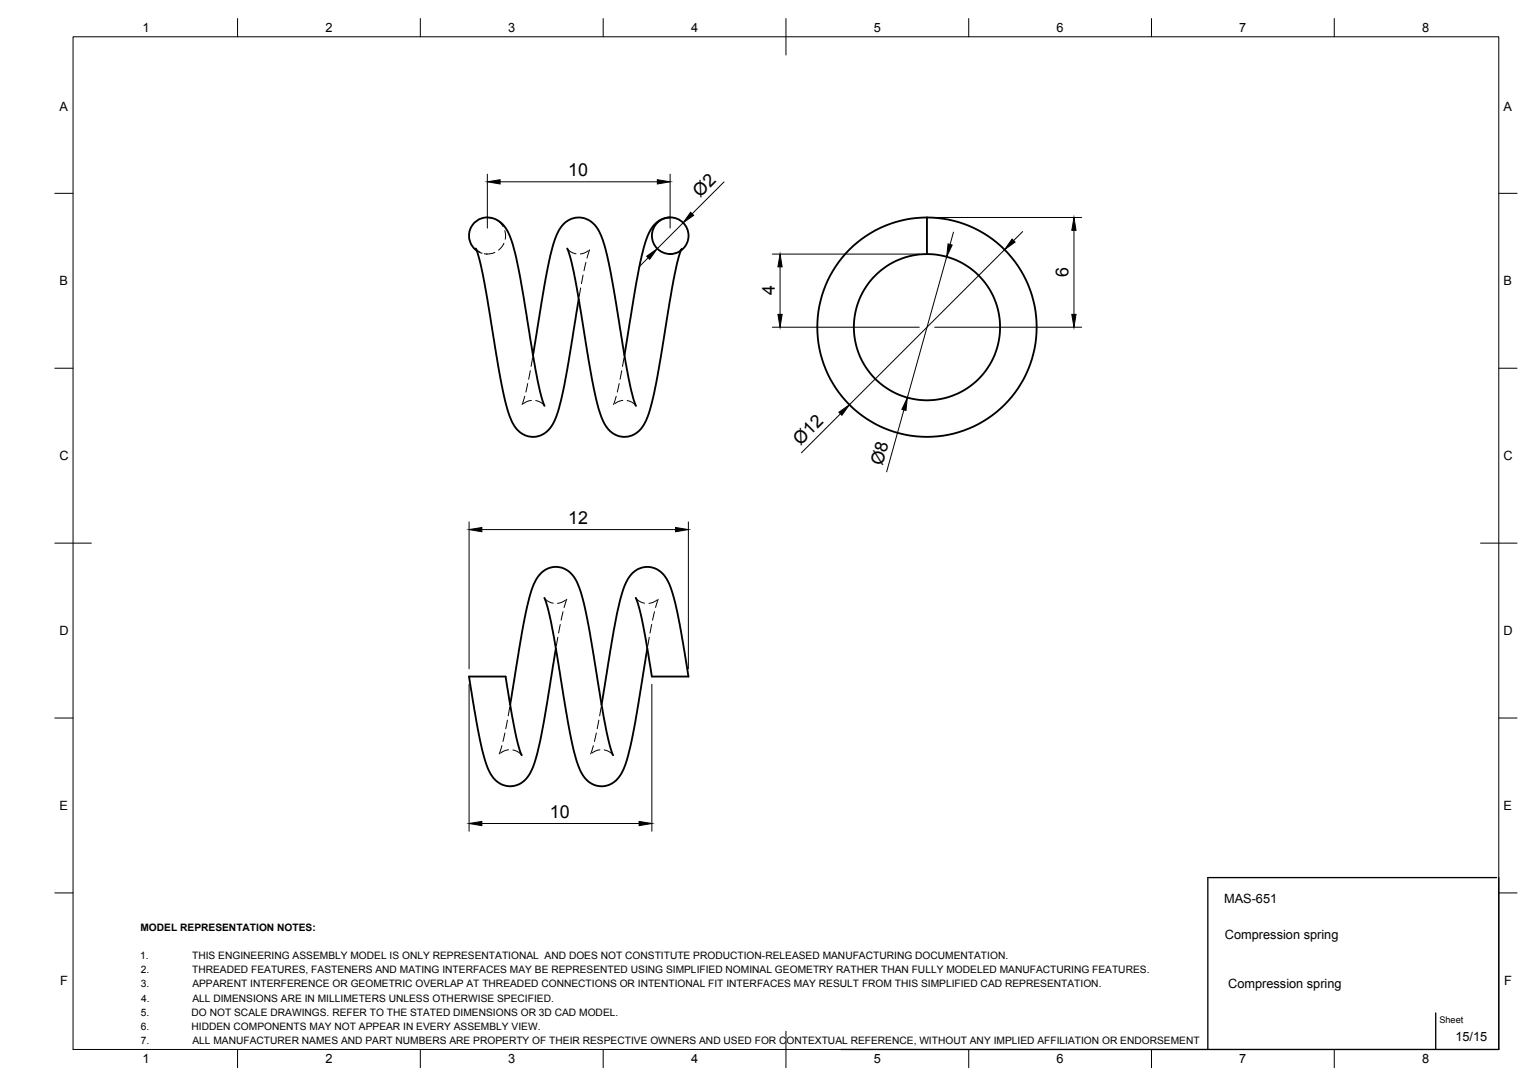
ISO-10303-21;
HEADER;
/* Generated by software containing ST-Developer
 * from STEP Tools, Inc. (www.steptools.com) 
 */

FILE_DESCRIPTION(
/* description */ ('Independent direct-acting normally-closed roller-plunger limit-switch
 CAD. Removable cover, insulated terminal supports, captured bus/conta
ct bridge, native Coil return spring, integral lower travel stop, reus
able instanced hardware and free roller. Manual geometric contact open
ing4mm; no snap-action/contact-force, electrical/current/voltage, envi
ronmental seal, safety-switch, wear, load or life certification. Exter
nal wiring and anchors omitted; fits and application engineering requi
red.'),
/* implementation_level */ '2;1');

FILE_NAME(
/* name */ 'Compression spring.step',
/* time_stamp */ '2026-11-08T07:32:43-08:00',
/* author */ (''),
/* organization */ (''),
/* preprocessor_version */ 'ST-DEVELOPER v20.2',
/* originating_system */ 'Autodesk Translation Framework v15.17.0.0',
/* authorisation */ '');

FILE_SCHEMA (('AUTOMOTIVE_DESIGN { 1 0 10303 214 3 1 1 }'));
ENDSEC;

DATA;
#10=MECHANICAL_DESIGN_GEOMETRIC_PRESENTATION_REPRESENTATION('',(#188),#36482);
#154=SHAPE_REPRESENTATION_RELATIONSHIP('SRR','None',#36567,#171);
#171=ADVANCED_BREP_SHAPE_REPRESENTATION('',(#205),#36477);
#188=STYLED_ITEM('',(#36660),#205);
#205=MANIFOLD_SOLID_BREP('Body1',#9779);
#228=B_SPLINE_SURFACE_WITH_KNOTS('',3,3,((#29315,#29316,#29317,#29318,#29319,
#29320,#29321,#29322,#29323,#29324,#29325,#29326,#29327,#29328,#29329,#29330,
#29331,#29332,#29333,#29334,#29335,#29336,#29337,#29338,#29339,#29340,#29341,
#29342,#29343),(#29344,#29345,#29346,#29347,#29348,#29349,#29350,#29351,
#29352,#29353,#29354,#29355,#29356,#29357,#29358,#29359,#29360,#29361,#29362,
#29363,#29364,#29365,#29366,#29367,#29368,#29369,#29370,#29371,#29372),
(#29373,#29374,#29375,#29376,#29377,#29378,#29379,#29380,#29381,#29382,
#29383,#29384,#29385,#29386,#29387,#29388,#29389,#29390,#29391,#29392,#29393,
#29394,#29395,#29396,#29397,#29398,#29399,#29400,#29401),(#29402,#29403,
#29404,#29405,#29406,#29407,#29408,#29409,#29410,#29411,#29412,#29413,#29414,
#29415,#29416,#29417,#29418,#29419,#29420,#29421,#29422,#29423,#29424,#29425,
#29426,#29427,#29428,#29429,#29430),(#29431,#29432,#29433,#29434,#29435,
#29436,#29437,#29438,#29439,#29440,#29441,#29442,#29443,#29444,#29445,#29446,
#29447,#29448,#29449,#29450,#29451,#29452,#29453,#29454,#29455,#29456,#29457,
#29458,#29459),(#29460,#29461,#29462,#29463,#29464,#29465,#29466,#29467,
#29468,#29469,#29470,#29471,#29472,#29473,#29474,#29475,#29476,#29477,#29478,
#29479,#29480,#29481,#29482,#29483,#29484,#29485,#29486,#29487,#29488),
(#29489,#29490,#29491,#29492,#29493,#29494,#29495,#29496,#29497,#29498,
#29499,#29500,#29501,#29502,#29503,#29504,#29505,#29506,#29507,#29508,#29509,
#29510,#29511,#29512,#29513,#29514,#29515,#29516,#29517),(#29518,#29519,
#29520,#29521,#29522,#29523,#29524,#29525,#29526,#29527,#29528,#29529,#29530,
#29531,#29532,#29533,#29534,#29535,#29536,#29537,#29538,#29539,#29540,#29541,
#29542,#29543,#29544,#29545,#29546),(#29547,#29548,#29549,#29550,#29551,
#29552,#29553,#29554,#29555,#29556,#29557,#29558,#29559,#29560,#29561,#29562,
#29563,#29564,#29565,#29566,#29567,#29568,#29569,#29570,#29571,#29572,#29573,
#29574,#29575),(#29576,#29577,#29578,#29579,#29580,#29581,#29582,#29583,
#29584,#29585,#29586,#29587,#29588,#29589,#29590,#29591,#29592,#29593,#29594,
#29595,#29596,#29597,#29598,#29599,#29600,#29601,#29602,#29603,#29604)),
 .UNSPECIFIED.,.T.,.F.,.F.,(4,1,1,1,1,1,1,4),(4,1,1,1,1,1,1,1,1,1,1,1,1,
1,1,1,1,1,1,1,1,1,1,1,1,1,4),(-3.14159265358979,-2.24399475256414,-1.34639685153848,
-0.448798950512828,0.448798950512828,1.34639685153848,2.24399475256414,
3.14159265358979),(0.,0.483321946706122,0.966643893412244,1.44996584011837,
1.93328778682449,2.41660973353061,2.89993168023673,3.38325362694285,3.86657557364898,
4.3498975203551,4.83321946706122,5.31654141376734,5.79986336047346,6.28318530717959,
6.76650725388571,7.24982920059183,7.73315114729795,8.21647309400407,8.6997950407102,
9.18311698741632,9.66643893412244,10.1497608808286,10.6330828275347,11.1164047742408,
11.5997267209469,12.083048667653,12.5663706143592),.UNSPECIFIED.);
#405=PLANE('',#10494);
#406=PLANE('',#10495);
#834=FACE_OUTER_BOUND('',#1431,.T.);
#835=FACE_OUTER_BOUND('',#1432,.T.);
#836=FACE_OUTER_BOUND('',#1433,.T.);
#1431=EDGE_LOOP('',(#8098,#8099,#8100,#8101));
#1432=EDGE_LOOP('',(#8102));
#1433=EDGE_LOOP('',(#8103));
#1711=CIRCLE('',#10492,0.1);
#1712=CIRCLE('',#10493,0.1);
#2241=B_SPLINE_CURVE_WITH_KNOTS('',3,(#29608,#29609,#29610,#29611,#29612,
#29613,#29614,#29615,#29616,#29617,#29618,#29619,#29620,#29621,#29622,#29623,
#29624,#29625,#29626,#29627,#29628,#29629,#29630,#29631,#29632,#29633,#29634,
#29635,#29636),.UNSPECIFIED.,.F.,.F.,(4,1,1,1,1,1,1,1,1,1,1,1,1,1,1,1,1,
1,1,1,1,1,1,1,1,1,4),(0.,0.483321946706122,0.966643893412244,1.44996584011837,
1.93328778682449,2.41660973353061,2.89993168023673,3.38325362694285,3.86657557364898,
4.3498975203551,4.83321946706122,5.31654141376734,5.79986336047346,6.28318530717959,
6.76650725388571,7.24982920059183,7.73315114729795,8.21647309400407,8.6997950407102,
9.18311698741632,9.66643893412244,10.1497608808286,10.6330828275347,11.1164047742408,
11.5997267209469,12.083048667653,12.5663706143592),.UNSPECIFIED.);
#4295=VERTEX_POINT('',#29605);
#4296=VERTEX_POINT('',#29607);
#5605=EDGE_CURVE('',#4295,#4295,#1711,.T.);
#5606=EDGE_CURVE('',#4295,#4296,#2241,.T.);
#5607=EDGE_CURVE('',#4296,#4296,#1712,.T.);
#8098=ORIENTED_EDGE('',*,*,#5605,.T.);
#8099=ORIENTED_EDGE('',*,*,#5606,.T.);
#8100=ORIENTED_EDGE('',*,*,#5607,.F.);
#8101=ORIENTED_EDGE('',*,*,#5606,.F.);
#8102=ORIENTED_EDGE('',*,*,#5607,.T.);
#8103=ORIENTED_EDGE('',*,*,#5605,.F.);
#9624=ADVANCED_FACE('',(#834),#228,.T.);
#9625=ADVANCED_FACE('',(#835),#405,.F.);
#9626=ADVANCED_FACE('',(#836),#406,.T.);
#9779=CLOSED_SHELL('',(#9624,#9625,#9626));
#10491=AXIS2_PLACEMENT_3D('',#29314,#12152,#12153);
#10492=AXIS2_PLACEMENT_3D('',#29606,#12154,#12155);
#10493=AXIS2_PLACEMENT_3D('',#29637,#12156,#12157);
#10494=AXIS2_PLACEMENT_3D('',#29638,#12158,#12159);
#10495=AXIS2_PLACEMENT_3D('',#29639,#12160,#12161);
#12152=DIRECTION('axis',(0.,0.,1.));
#12153=DIRECTION('refdir',(1.,0.,0.));
#12154=DIRECTION('center_axis',(0.,0.,-1.));
#12155=DIRECTION('ref_axis',(-1.,0.,0.));
#12156=DIRECTION('center_axis',(4.89858719658941E-16,0.,-1.));
#12157=DIRECTION('ref_axis',(-1.,0.,-4.89858719658941E-16));
#12158=DIRECTION('center_axis',(-4.89858719658941E-16,0.,1.));
#12159=DIRECTION('ref_axis',(1.,0.,4.89858719658941E-16));
#12160=DIRECTION('center_axis',(0.,0.,1.));
#12161=DIRECTION('ref_axis',(1.,0.,0.));
#29314=CARTESIAN_POINT('',(0.,0.,0.));
#29315=CARTESIAN_POINT('Ctrl Pts',(0.6,-1.22464679914735E-17,0.));
#29316=CARTESIAN_POINT('Ctrl Pts',(0.6,0.0128205128205128,-0.0966643893412244));
#29317=CARTESIAN_POINT('Ctrl Pts',(0.552422075024677,0.0384615384615385,
-0.289907779312461));
#29318=CARTESIAN_POINT('Ctrl Pts',(0.354387423761003,0.0769230769230769,
-0.513439446520879));
#29319=CARTESIAN_POINT('Ctrl Pts',(0.0752027553952744,0.115384615384615,
-0.619312950390957));
#29320=CARTESIAN_POINT('Ctrl Pts',(-0.221227750860346,0.153846153846154,
-0.583326335743102));
#29321=CARTESIAN_POINT('Ctrl Pts',(-0.466969125257516,0.192307692307692,
-0.413698471057249));
#29322=CARTESIAN_POINT('Ctrl Pts',(-0.605737625154647,0.230769230769231,
-0.149301246402526));
#29323=CARTESIAN_POINT('Ctrl Pts',(-0.605736940333524,0.269230769230769,
0.14930101675222));
#29324=CARTESIAN_POINT('Ctrl Pts',(-0.466970187413293,0.307692307692308,
0.413699286558057));
#29325=CARTESIAN_POINT('Ctrl Pts',(-0.221225725123394,0.346153846153846,
0.583324484886018));
#29326=CARTESIAN_POINT('Ctrl Pts',(0.0751986583056162,0.384615384615385,
0.619316856641734));
#29327=CARTESIAN_POINT('Ctrl Pts',(0.354396045955746,0.423076923076923,
0.513431304005641));
#29328=CARTESIAN_POINT('Ctrl Pts',(0.55240551470084,0.461538461538462,0.289924779022985));
#29329=CARTESIAN_POINT('Ctrl Pts',(0.623865568763842,0.5,3.99584594159288E-16));
#29330=CARTESIAN_POINT('Ctrl Pts',(0.552405514700841,0.538461538461539,
-0.289924779022984));
#29331=CARTESIAN_POINT('Ctrl Pts',(0.354396045955747,0.576923076923077,
-0.513431304005641));
#29332=CARTESIAN_POINT('Ctrl Pts',(0.0751986583056171,0.615384615384616,
-0.619316856641735));
#29333=CARTESIAN_POINT('Ctrl Pts',(-0.221225725123393,0.653846153846154,
-0.583324484886017));
#29334=CARTESIAN_POINT('Ctrl Pts',(-0.466970187413293,0.692307692307693,
-0.413699286558058));
#29335=CARTESIAN_POINT('Ctrl Pts',(-0.605736940333523,0.730769230769231,
-0.149301016752221));
#29336=CARTESIAN_POINT('Ctrl Pts',(-0.605737625154647,0.769230769230769,
0.149301246402525));
#29337=CARTESIAN_POINT('Ctrl Pts',(-0.466969125257516,0.807692307692308,
0.41369847105725));
#29338=CARTESIAN_POINT('Ctrl Pts',(-0.221227750860347,0.846153846153846,
0.583326335743102));
#29339=CARTESIAN_POINT('Ctrl Pts',(0.0752027553952735,0.884615384615385,
0.619312950390957));
#29340=CARTESIAN_POINT('Ctrl Pts',(0.354387423761003,0.923076923076923,
0.513439446520879));
#29341=CARTESIAN_POINT('Ctrl Pts',(0.552422075024676,0.961538461538462,
0.289907779312462));
#29342=CARTESIAN_POINT('Ctrl Pts',(0.6,0.987179487179487,0.096664389341225));
#29343=CARTESIAN_POINT('Ctrl Pts',(0.6,1.,2.93915231795365E-16));
#29344=CARTESIAN_POINT('Ctrl Pts',(0.6,-0.0299199300341885,0.));
#29345=CARTESIAN_POINT('Ctrl Pts',(0.6,-0.0170994172136757,-0.09670823080664));
#29346=CARTESIAN_POINT('Ctrl Pts',(0.552433668035603,0.00854160842734991,
-0.289889597147613));
#29347=CARTESIAN_POINT('Ctrl Pts',(0.354391049739123,0.0470031468888885,
-0.513458052176708));
#29348=CARTESIAN_POINT('Ctrl Pts',(0.0752046939357531,0.0854646853504268,
-0.619317061421753));
#29349=CARTESIAN_POINT('Ctrl Pts',(-0.221231470738224,0.123926223811965,
-0.583337632633336));
#29350=CARTESIAN_POINT('Ctrl Pts',(-0.466975962510102,0.162387762273504,
-0.413703477287484));
#29351=CARTESIAN_POINT('Ctrl Pts',(-0.605746831003298,0.200849300735043,
-0.149304082326356));
#29352=CARTESIAN_POINT('Ctrl Pts',(-0.605746010438017,0.239310839196581,
0.149303548319889));
#29353=CARTESIAN_POINT('Ctrl Pts',(-0.466977235204714,0.277772377658119,
0.413705373558643));
#29354=CARTESIAN_POINT('Ctrl Pts',(-0.221229043462903,0.316233916119658,
0.58333332852287));
#29355=CARTESIAN_POINT('Ctrl Pts',(0.0751997847274774,0.354695454581196,
0.619326143478273));
#29356=CARTESIAN_POINT('Ctrl Pts',(0.35440138101164,0.393156993042734,0.513439044221362));
#29357=CARTESIAN_POINT('Ctrl Pts',(0.552413825150628,0.431618531504273,
0.289929135658685));
#29358=CARTESIAN_POINT('Ctrl Pts',(0.623874957033007,0.470080069965812,
3.99584594159288E-16));
#29359=CARTESIAN_POINT('Ctrl Pts',(0.552413825150628,0.50854160842735,-0.289929135658685));
#29360=CARTESIAN_POINT('Ctrl Pts',(0.354401381011641,0.547003146888889,
-0.513439044221361));
#29361=CARTESIAN_POINT('Ctrl Pts',(0.0751997847274784,0.585464685350427,
-0.619326143478273));
#29362=CARTESIAN_POINT('Ctrl Pts',(-0.221229043462903,0.623926223811966,
-0.583333328522871));
#29363=CARTESIAN_POINT('Ctrl Pts',(-0.466977235204713,0.662387762273504,
-0.413705373558643));
#29364=CARTESIAN_POINT('Ctrl Pts',(-0.605746010438017,0.700849300735043,
-0.14930354831989));
#29365=CARTESIAN_POINT('Ctrl Pts',(-0.605746831003298,0.73931083919658,
0.149304082326356));
#29366=CARTESIAN_POINT('Ctrl Pts',(-0.466975962510103,0.77777237765812,
0.413703477287484));
#29367=CARTESIAN_POINT('Ctrl Pts',(-0.221231470738224,0.816233916119658,
0.583337632633336));
#29368=CARTESIAN_POINT('Ctrl Pts',(0.0752046939357522,0.854695454581196,
0.619317061421752));
#29369=CARTESIAN_POINT('Ctrl Pts',(0.354391049739122,0.893156993042734,
0.513458052176709));
#29370=CARTESIAN_POINT('Ctrl Pts',(0.552433668035603,0.931618531504273,
0.289889597147614));
#29371=CARTESIAN_POINT('Ctrl Pts',(0.6,0.957259557145299,0.0967082308066405));
#29372=CARTESIAN_POINT('Ctrl Pts',(0.6,0.970080069965812,2.93915231795365E-16));
#29373=CARTESIAN_POINT('Ctrl Pts',(0.57140278473399,-0.0895099491231781,
0.));
#29374=CARTESIAN_POINT('Ctrl Pts',(0.57140278473399,-0.0766894363026653,
-0.0920388134316465));
#29375=CARTESIAN_POINT('Ctrl Pts',(0.526087666325587,-0.0510484106616395,
-0.27609779977643));
#29376=CARTESIAN_POINT('Ctrl Pts',(0.337495083246531,-0.0125868722001011,
-0.488960092834314));
#29377=CARTESIAN_POINT('Ctrl Pts',(0.071617628135789,0.0258746662614374,
-0.589793519606227));
#29378=CARTESIAN_POINT('Ctrl Pts',(-0.210682030750213,0.064336204722976,
-0.555519091361673));
#29379=CARTESIAN_POINT('Ctrl Pts',(-0.444709568341539,0.102797743184514,
-0.393978668020424));
#29380=CARTESIAN_POINT('Ctrl Pts',(-0.57686308879389,0.141259281646053,
-0.142184059267368));
#29381=CARTESIAN_POINT('Ctrl Pts',(-0.576862493445414,0.179720820107591,
0.142183967988976));
#29382=CARTESIAN_POINT('Ctrl Pts',(-0.444710491725475,0.21818235856913,
0.39397899216129));
#29383=CARTESIAN_POINT('Ctrl Pts',(-0.21068026967806,0.256643897030668,
0.555518355836033));
#29384=CARTESIAN_POINT('Ctrl Pts',(0.0716140663354809,0.295105435492207,
0.589795072696736));
#29385=CARTESIAN_POINT('Ctrl Pts',(0.337502578941879,0.333566973953745,
0.488956887495931));
#29386=CARTESIAN_POINT('Ctrl Pts',(0.526073269626597,0.372028512415283,
0.276104552814102));
#29387=CARTESIAN_POINT('Ctrl Pts',(0.59412694151864,0.410490050876822,3.42501080707961E-16));
#29388=CARTESIAN_POINT('Ctrl Pts',(0.526073269626597,0.448951589338361,
-0.276104552814101));
#29389=CARTESIAN_POINT('Ctrl Pts',(0.33750257894188,0.487413127799899,-0.488956887495931));
#29390=CARTESIAN_POINT('Ctrl Pts',(0.0716140663354816,0.525874666261437,
-0.589795072696736));
#29391=CARTESIAN_POINT('Ctrl Pts',(-0.21068026967806,0.564336204722976,
-0.555518355836033));
#29392=CARTESIAN_POINT('Ctrl Pts',(-0.444710491725474,0.602797743184515,
-0.393978992161291));
#29393=CARTESIAN_POINT('Ctrl Pts',(-0.576862493445414,0.641259281646054,
-0.142183967988976));
#29394=CARTESIAN_POINT('Ctrl Pts',(-0.576863088793891,0.679720820107591,
0.142184059267367));
#29395=CARTESIAN_POINT('Ctrl Pts',(-0.44470956834154,0.718182358569131,
0.393978668020424));
#29396=CARTESIAN_POINT('Ctrl Pts',(-0.210682030750213,0.756643897030668,
0.555519091361672));
#29397=CARTESIAN_POINT('Ctrl Pts',(0.0716176281357881,0.795105435492208,
0.589793519606227));
#29398=CARTESIAN_POINT('Ctrl Pts',(0.33749508324653,0.833566973953744,0.488960092834314));
#29399=CARTESIAN_POINT('Ctrl Pts',(0.526087666325587,0.872028512415284,
0.276097799776431));
#29400=CARTESIAN_POINT('Ctrl Pts',(0.57140278473399,0.89766953805631,0.092038813431647));
#29401=CARTESIAN_POINT('Ctrl Pts',(0.57140278473399,0.910490050876822,2.79906636539346E-16));
#29402=CARTESIAN_POINT('Ctrl Pts',(0.474553946216323,-0.111561765583155,
0.));
#29403=CARTESIAN_POINT('Ctrl Pts',(0.474553946216323,-0.0987412527626418,
-0.0764564796257483));
#29404=CARTESIAN_POINT('Ctrl Pts',(0.436924085441389,-0.0731002271216164,
-0.229293819423993));
#29405=CARTESIAN_POINT('Ctrl Pts',(0.28029344651323,-0.0346386886600778,
-0.406092197111352));
#29406=CARTESIAN_POINT('Ctrl Pts',(0.0594797119051372,0.00382284980146056,
-0.489829229563544));
#29407=CARTESIAN_POINT('Ctrl Pts',(-0.174974371163627,0.0422843882629991,
-0.461366967583472));
#29408=CARTESIAN_POINT('Ctrl Pts',(-0.369337104437002,0.0807459267245375,
-0.327204006955578));
#29409=CARTESIAN_POINT('Ctrl Pts',(-0.479092464392592,0.119207465186076,
-0.118085979220413));
#29410=CARTESIAN_POINT('Ctrl Pts',(-0.479091915422023,0.157669003647615,
0.118085781150671));
#29411=CARTESIAN_POINT('Ctrl Pts',(-0.369337955888923,0.196130542109153,
0.327204710311264));
#29412=CARTESIAN_POINT('Ctrl Pts',(-0.17497274727977,0.234592080570691,
0.461365371232019));
#29413=CARTESIAN_POINT('Ctrl Pts',(0.0594764275706395,0.27305361903223,
0.489832598580241));
#29414=CARTESIAN_POINT('Ctrl Pts',(0.280300358290614,0.311515157493768,
0.406085170317839));
#29415=CARTESIAN_POINT('Ctrl Pts',(0.436910810251582,0.349976695955307,
0.229308481892446));
#29416=CARTESIAN_POINT('Ctrl Pts',(0.493430286203431,0.388438234416845,
3.28230202345129E-16));
#29417=CARTESIAN_POINT('Ctrl Pts',(0.436910810251583,0.426899772878384,
-0.229308481892445));
#29418=CARTESIAN_POINT('Ctrl Pts',(0.280300358290614,0.465361311339922,
-0.406085170317838));
#29419=CARTESIAN_POINT('Ctrl Pts',(0.0594764275706403,0.503822849801461,
-0.489832598580241));
#29420=CARTESIAN_POINT('Ctrl Pts',(-0.17497274727977,0.542284388262999,
-0.461365371232019));
#29421=CARTESIAN_POINT('Ctrl Pts',(-0.369337955888923,0.580745926724537,
-0.327204710311264));
#29422=CARTESIAN_POINT('Ctrl Pts',(-0.479091915422023,0.619207465186076,
-0.118085781150672));
#29423=CARTESIAN_POINT('Ctrl Pts',(-0.479092464392592,0.657669003647615,
0.118085979220413));
#29424=CARTESIAN_POINT('Ctrl Pts',(-0.369337104437003,0.696130542109153,
0.327204006955579));
#29425=CARTESIAN_POINT('Ctrl Pts',(-0.174974371163627,0.734592080570691,
0.461366967583471));
#29426=CARTESIAN_POINT('Ctrl Pts',(0.0594797119051365,0.773053619032229,
0.489829229563544));
#29427=CARTESIAN_POINT('Ctrl Pts',(0.280293446513229,0.811515157493768,
0.406092197111352));
#29428=CARTESIAN_POINT('Ctrl Pts',(0.436924085441388,0.849976695955308,
0.229293819423994));
#29429=CARTESIAN_POINT('Ctrl Pts',(0.474553946216323,0.875617721596332,
0.0764564796257487));
#29430=CARTESIAN_POINT('Ctrl Pts',(0.474553946216323,0.888438234416845,
2.32464388502626E-16));
#29431=CARTESIAN_POINT('Ctrl Pts',(0.396775149169774,-0.0496835058675068,
0.));
#29432=CARTESIAN_POINT('Ctrl Pts',(0.396775149169774,-0.036862993046994,
-0.0639325270983766));
#29433=CARTESIAN_POINT('Ctrl Pts',(0.365314671027668,-0.0112219674059683,
-0.19170987675844));
#29434=CARTESIAN_POINT('Ctrl Pts',(0.23435429480531,0.0272395710555702,
-0.339537237215488));
#29435=CARTESIAN_POINT('Ctrl Pts',(0.0497313786444746,0.0657011095171087,
-0.409547504928549));
#29436=CARTESIAN_POINT('Ctrl Pts',(-0.146296899267444,0.104162647978647,
-0.385751347000212));
#29437=CARTESIAN_POINT('Ctrl Pts',(-0.308804333876165,0.142624186440185,
-0.273576498871778));
#29438=CARTESIAN_POINT('Ctrl Pts',(-0.400571315183775,0.181085724901724,
-0.0987322989296554));
#29439=CARTESIAN_POINT('Ctrl Pts',(-0.400570833992816,0.219547263363262,
0.098732083557009));
#29440=CARTESIAN_POINT('Ctrl Pts',(-0.308805080202088,0.258008801824801,
0.273577263668698));
#29441=CARTESIAN_POINT('Ctrl Pts',(-0.146295475879243,0.296470340286339,
0.385749611149152));
#29442=CARTESIAN_POINT('Ctrl Pts',(0.0497284998160722,0.334931878747878,
0.409551168080821));
#29443=CARTESIAN_POINT('Ctrl Pts',(0.234360353208027,0.373393417209416,
0.339529585460424));
#29444=CARTESIAN_POINT('Ctrl Pts',(0.365303034882358,0.411854955670955,
0.19172582146083));
#29445=CARTESIAN_POINT('Ctrl Pts',(0.412559215796984,0.450316494132494,
2.28334053805307E-16));
#29446=CARTESIAN_POINT('Ctrl Pts',(0.365303034882358,0.488778032594032,
-0.191725821460829));
#29447=CARTESIAN_POINT('Ctrl Pts',(0.234360353208027,0.52723957105557,-0.339529585460423));
#29448=CARTESIAN_POINT('Ctrl Pts',(0.049728499816073,0.565701109517109,
-0.409551168080821));
#29449=CARTESIAN_POINT('Ctrl Pts',(-0.146295475879243,0.604162647978647,
-0.385749611149151));
#29450=CARTESIAN_POINT('Ctrl Pts',(-0.308805080202087,0.642624186440186,
-0.273577263668699));
#29451=CARTESIAN_POINT('Ctrl Pts',(-0.400570833992816,0.681085724901724,
-0.0987320835570092));
#29452=CARTESIAN_POINT('Ctrl Pts',(-0.400571315183774,0.719547263363262,
0.0987322989296545));
#29453=CARTESIAN_POINT('Ctrl Pts',(-0.308804333876166,0.758008801824802,
0.273576498871779));
#29454=CARTESIAN_POINT('Ctrl Pts',(-0.146296899267444,0.79647034028634,
0.385751347000211));
#29455=CARTESIAN_POINT('Ctrl Pts',(0.0497313786444738,0.834931878747878,
0.409547504928549));
#29456=CARTESIAN_POINT('Ctrl Pts',(0.234354294805309,0.873393417209416,
0.339537237215489));
#29457=CARTESIAN_POINT('Ctrl Pts',(0.365314671027668,0.911854955670954,
0.191709876758441));
#29458=CARTESIAN_POINT('Ctrl Pts',(0.396775149169774,0.937495981311981,
0.0639325270983769));
#29459=CARTESIAN_POINT('Ctrl Pts',(0.396775149169774,0.950316494132494,
1.94363766564791E-16));
#29460=CARTESIAN_POINT('Ctrl Pts',(0.396939270424005,0.0496169828764393,
0.));
#29461=CARTESIAN_POINT('Ctrl Pts',(0.396939270424005,0.0624374956969522,
-0.0639374232798038));
#29462=CARTESIAN_POINT('Ctrl Pts',(0.36546008089603,0.0880785213379777,
-0.191798112042878));
#29463=CARTESIAN_POINT('Ctrl Pts',(0.234449450409805,0.126540059799516,
-0.339668537739251));
#29464=CARTESIAN_POINT('Ctrl Pts',(0.049750996607657,0.165001598261055,
-0.409714888680431));
#29465=CARTESIAN_POINT('Ctrl Pts',(-0.146355584839357,0.203463136722593,
-0.385905355800823));
#29466=CARTESIAN_POINT('Ctrl Pts',(-0.308928706451725,0.241924675184131,
-0.273687199853259));
#29467=CARTESIAN_POINT('Ctrl Pts',(-0.400732481863726,0.28038621364567,
-0.0987717444550605));
#29468=CARTESIAN_POINT('Ctrl Pts',(-0.400732067194017,0.318847752107208,
0.0987716785889419));
#29469=CARTESIAN_POINT('Ctrl Pts',(-0.308929349603364,0.357309290568747,
0.273687433751705));
#29470=CARTESIAN_POINT('Ctrl Pts',(-0.146354358224513,0.395770829030285,
0.385904825042549));
#29471=CARTESIAN_POINT('Ctrl Pts',(0.0497485157569321,0.434232367491824,
0.40971600936184));
#29472=CARTESIAN_POINT('Ctrl Pts',(0.234454671281171,0.472693905953362,
0.339666223345759));
#29473=CARTESIAN_POINT('Ctrl Pts',(0.365450053365557,0.511155444414901,
0.191802985182395));
#29474=CARTESIAN_POINT('Ctrl Pts',(0.412725251465001,0.549616982876439,
3.13959323982298E-16));
#29475=CARTESIAN_POINT('Ctrl Pts',(0.365450053365557,0.588078521337977,
-0.191802985182395));
#29476=CARTESIAN_POINT('Ctrl Pts',(0.234454671281172,0.626540059799516,
-0.339666223345758));
#29477=CARTESIAN_POINT('Ctrl Pts',(0.0497485157569325,0.665001598261056,
-0.409716009361841));
#29478=CARTESIAN_POINT('Ctrl Pts',(-0.146354358224513,0.703463136722593,
-0.385904825042548));
#29479=CARTESIAN_POINT('Ctrl Pts',(-0.308929349603364,0.741924675184131,
-0.273687433751706));
#29480=CARTESIAN_POINT('Ctrl Pts',(-0.400732067194016,0.78038621364567,
-0.0987716785889423));
#29481=CARTESIAN_POINT('Ctrl Pts',(-0.400732481863727,0.818847752107209,
0.09877174445506));
#29482=CARTESIAN_POINT('Ctrl Pts',(-0.308928706451726,0.857309290568746,
0.273687199853259));
#29483=CARTESIAN_POINT('Ctrl Pts',(-0.146355584839357,0.895770829030286,
0.385905355800823));
#29484=CARTESIAN_POINT('Ctrl Pts',(0.0497509966076566,0.934232367491823,
0.409714888680431));
#29485=CARTESIAN_POINT('Ctrl Pts',(0.234449450409805,0.972693905953362,
0.339668537739251));
#29486=CARTESIAN_POINT('Ctrl Pts',(0.36546008089603,1.0111554444149,0.191798112042878));
#29487=CARTESIAN_POINT('Ctrl Pts',(0.396939270424005,1.03679647005593,0.0639374232798042));
#29488=CARTESIAN_POINT('Ctrl Pts',(0.396939270424005,1.04961698287644,1.94444162792257E-16));
#29489=CARTESIAN_POINT('Ctrl Pts',(0.474480121999477,0.111725197096412,
0.));
#29490=CARTESIAN_POINT('Ctrl Pts',(0.474480121999477,0.124545709916925,
-0.0764586335789696));
#29491=CARTESIAN_POINT('Ctrl Pts',(0.436859829833703,0.150186735557951,
-0.229252323181468));
#29492=CARTESIAN_POINT('Ctrl Pts',(0.28025100438353,0.188648274019489,-0.406034984914813));
#29493=CARTESIAN_POINT('Ctrl Pts',(0.0594710800733114,0.227109812481028,
-0.489754346320688));
#29494=CARTESIAN_POINT('Ctrl Pts',(-0.174948343135337,0.265571350942566,
-0.461298814622112));
#29495=CARTESIAN_POINT('Ctrl Pts',(-0.369281839162736,0.304032889404105,
-0.327154709430175));
#29496=CARTESIAN_POINT('Ctrl Pts',(-0.479020883931678,0.342494427865643,
-0.118068517820842));
#29497=CARTESIAN_POINT('Ctrl Pts',(-0.47902029155056,0.380955966327182,
0.118068222258303));
#29498=CARTESIAN_POINT('Ctrl Pts',(-0.369282757944306,0.41941750478872,
0.327155758983302));
#29499=CARTESIAN_POINT('Ctrl Pts',(-0.17494659084079,0.457879043250258,
0.461296432432969));
#29500=CARTESIAN_POINT('Ctrl Pts',(0.0594675360258692,0.496340581711797,
0.489759373275717));
#29501=CARTESIAN_POINT('Ctrl Pts',(0.280258462718537,0.534802120173335,
0.406024477645537));
#29502=CARTESIAN_POINT('Ctrl Pts',(0.436845504891309,0.573263658634874,
0.22927420538536));
#29503=CARTESIAN_POINT('Ctrl Pts',(0.493356533724516,0.611725197096412,
3.99584594159288E-16));
#29504=CARTESIAN_POINT('Ctrl Pts',(0.43684550489131,0.650186735557951,-0.229274205385359));
#29505=CARTESIAN_POINT('Ctrl Pts',(0.280258462718538,0.688648274019488,
-0.406024477645536));
#29506=CARTESIAN_POINT('Ctrl Pts',(0.0594675360258697,0.727109812481028,
-0.489759373275717));
#29507=CARTESIAN_POINT('Ctrl Pts',(-0.174946590840789,0.765571350942565,
-0.461296432432969));
#29508=CARTESIAN_POINT('Ctrl Pts',(-0.369282757944306,0.804032889404106,
-0.327155758983302));
#29509=CARTESIAN_POINT('Ctrl Pts',(-0.47902029155056,0.842494427865642,
-0.118068222258304));
#29510=CARTESIAN_POINT('Ctrl Pts',(-0.479020883931677,0.880955966327181,
0.118068517820842));
#29511=CARTESIAN_POINT('Ctrl Pts',(-0.369281839162738,0.91941750478872,
0.327154709430175));
#29512=CARTESIAN_POINT('Ctrl Pts',(-0.174948343135337,0.957879043250258,
0.461298814622112));
#29513=CARTESIAN_POINT('Ctrl Pts',(0.0594710800733105,0.996340581711796,
0.489754346320688));
#29514=CARTESIAN_POINT('Ctrl Pts',(0.28025100438353,1.03480212017334,0.406034984914813));
#29515=CARTESIAN_POINT('Ctrl Pts',(0.436859829833702,1.07326365863487,0.229252323181468));
#29516=CARTESIAN_POINT('Ctrl Pts',(0.474480121999477,1.0989046842759,0.0764586335789701));
#29517=CARTESIAN_POINT('Ctrl Pts',(0.474480121999477,1.11172519709641,2.32428225066282E-16));
#29518=CARTESIAN_POINT('Ctrl Pts',(0.571396374369977,0.0893939875669938,
0.));
#29519=CARTESIAN_POINT('Ctrl Pts',(0.571396374369977,0.102214500387507,
-0.0920304506152003));
#29520=CARTESIAN_POINT('Ctrl Pts',(0.526079825991483,0.127855526028532,
-0.27609774238039));
#29521=CARTESIAN_POINT('Ctrl Pts',(0.337490690748289,0.166317064490071,
-0.488951496511335));
#29522=CARTESIAN_POINT('Ctrl Pts',(0.0716165005604001,0.204778602951609,
-0.589786215561319));
#29523=CARTESIAN_POINT('Ctrl Pts',(-0.210679045222389,0.243240141413148,
-0.555510970358107));
#29524=CARTESIAN_POINT('Ctrl Pts',(-0.444703436119133,0.281701679874686,
-0.393973411075695));
#29525=CARTESIAN_POINT('Ctrl Pts',(-0.576855077960488,0.320163218336225,
-0.142181989990421));
#29526=CARTESIAN_POINT('Ctrl Pts',(-0.576854505315029,0.358624756797763,
0.142181949601214));
#29527=CARTESIAN_POINT('Ctrl Pts',(-0.444704324290748,0.397086295259301,
0.393973554508792));
#29528=CARTESIAN_POINT('Ctrl Pts',(-0.210677351306959,0.43554783372084,
0.555510645023163));
#29529=CARTESIAN_POINT('Ctrl Pts',(0.0716130745857797,0.474009372182378,
0.589786903242894));
#29530=CARTESIAN_POINT('Ctrl Pts',(0.337497900602802,0.512470910643917,
0.48895010790376));
#29531=CARTESIAN_POINT('Ctrl Pts',(0.526065978296192,0.550932449105455,
0.276100726868827));
#29532=CARTESIAN_POINT('Ctrl Pts',(0.594118706507634,0.589393987566993,
4.28126350884951E-16));
#29533=CARTESIAN_POINT('Ctrl Pts',(0.526065978296193,0.627855526028533,
-0.276100726868826));
#29534=CARTESIAN_POINT('Ctrl Pts',(0.337497900602802,0.66631706449007,-0.48895010790376));
#29535=CARTESIAN_POINT('Ctrl Pts',(0.0716130745857805,0.70477860295161,
-0.589786903242894));
#29536=CARTESIAN_POINT('Ctrl Pts',(-0.210677351306959,0.743240141413148,
-0.555510645023163));
#29537=CARTESIAN_POINT('Ctrl Pts',(-0.444704324290748,0.781701679874686,
-0.393973554508792));
#29538=CARTESIAN_POINT('Ctrl Pts',(-0.576854505315029,0.820163218336225,
-0.142181949601214));
#29539=CARTESIAN_POINT('Ctrl Pts',(-0.576855077960488,0.858624756797763,
0.14218198999042));
#29540=CARTESIAN_POINT('Ctrl Pts',(-0.444703436119134,0.897086295259303,
0.393973411075695));
#29541=CARTESIAN_POINT('Ctrl Pts',(-0.210679045222389,0.935547833720839,
0.555510970358107));
#29542=CARTESIAN_POINT('Ctrl Pts',(0.0716165005603993,0.97400937218238,
0.589786215561319));
#29543=CARTESIAN_POINT('Ctrl Pts',(0.337490690748288,1.01247091064392,0.488951496511335));
#29544=CARTESIAN_POINT('Ctrl Pts',(0.526079825991483,1.05093244910546,0.27609774238039));
#29545=CARTESIAN_POINT('Ctrl Pts',(0.571396374369977,1.07657347474648,0.0920304506152009));
#29546=CARTESIAN_POINT('Ctrl Pts',(0.571396374369977,1.08939398756699,2.79903496366638E-16));
#29547=CARTESIAN_POINT('Ctrl Pts',(0.6,0.0299199300341885,0.));
#29548=CARTESIAN_POINT('Ctrl Pts',(0.6,0.0427404428547013,-0.0967139473831177));
#29549=CARTESIAN_POINT('Ctrl Pts',(0.552435179671515,0.068381468495727,
-0.289887226338725));
#29550=CARTESIAN_POINT('Ctrl Pts',(0.354391522537672,0.106843006957265,
-0.513460478205433));
#29551=CARTESIAN_POINT('Ctrl Pts',(0.0752049467059282,0.145304545418804,
-0.619317597467292));
#29552=CARTESIAN_POINT('Ctrl Pts',(-0.22123195578055,0.183766083880342,
-0.583339105657478));
#29553=CARTESIAN_POINT('Ctrl Pts',(-0.46697685403316,0.222227622341881,
-0.413704130059871));
#29554=CARTESIAN_POINT('Ctrl Pts',(-0.60574803137234,0.260689160803419,
-0.149304452108144));
#29555=CARTESIAN_POINT('Ctrl Pts',(-0.605747193107107,0.299150699264958,
0.149303878416068));
#29556=CARTESIAN_POINT('Ctrl Pts',(-0.466978154180352,0.337612237726497,
0.41370616725484));
#29557=CARTESIAN_POINT('Ctrl Pts',(-0.221229476147838,0.376073776188034,
0.58333448166239));
#29558=CARTESIAN_POINT('Ctrl Pts',(0.0751999316038799,0.414535314649573,
0.619327354407488));
#29559=CARTESIAN_POINT('Ctrl Pts',(0.354402076660262,0.452996853111111,
0.513440053483591));
#29560=CARTESIAN_POINT('Ctrl Pts',(0.552414908766819,0.49145839157265,0.28992970372914));
#29561=CARTESIAN_POINT('Ctrl Pts',(0.623876181188225,0.529919930034188,
3.71042837433625E-16));
#29562=CARTESIAN_POINT('Ctrl Pts',(0.552414908766819,0.568381468495727,
-0.289929703729139));
#29563=CARTESIAN_POINT('Ctrl Pts',(0.354402076660263,0.606843006957265,
-0.51344005348359));
#29564=CARTESIAN_POINT('Ctrl Pts',(0.0751999316038808,0.645304545418805,
-0.619327354407488));
#29565=CARTESIAN_POINT('Ctrl Pts',(-0.221229476147837,0.683766083880342,
-0.583334481662391));
#29566=CARTESIAN_POINT('Ctrl Pts',(-0.466978154180352,0.722227622341881,
-0.41370616725484));
#29567=CARTESIAN_POINT('Ctrl Pts',(-0.605747193107107,0.760689160803419,
-0.149303878416068));
#29568=CARTESIAN_POINT('Ctrl Pts',(-0.60574803137234,0.799150699264958,
0.149304452108143));
#29569=CARTESIAN_POINT('Ctrl Pts',(-0.466976854033161,0.837612237726496,
0.41370413005987));
#29570=CARTESIAN_POINT('Ctrl Pts',(-0.22123195578055,0.876073776188035,
0.583339105657478));
#29571=CARTESIAN_POINT('Ctrl Pts',(0.0752049467059273,0.914535314649573,
0.619317597467291));
#29572=CARTESIAN_POINT('Ctrl Pts',(0.354391522537671,0.952996853111112,
0.513460478205434));
#29573=CARTESIAN_POINT('Ctrl Pts',(0.552435179671515,0.99145839157265,0.289887226338726));
#29574=CARTESIAN_POINT('Ctrl Pts',(0.6,1.01709941721368,0.0967139473831183));
#29575=CARTESIAN_POINT('Ctrl Pts',(0.6,1.02991993003419,2.93915231795365E-16));
#29576=CARTESIAN_POINT('Ctrl Pts',(0.6,1.22464679914735E-17,0.));
#29577=CARTESIAN_POINT('Ctrl Pts',(0.6,0.0128205128205128,-0.0966643893412244));
#29578=CARTESIAN_POINT('Ctrl Pts',(0.552422075024677,0.0384615384615385,
-0.289907779312461));
#29579=CARTESIAN_POINT('Ctrl Pts',(0.354387423761003,0.076923076923077,
-0.513439446520879));
#29580=CARTESIAN_POINT('Ctrl Pts',(0.0752027553952744,0.115384615384615,
-0.619312950390957));
#29581=CARTESIAN_POINT('Ctrl Pts',(-0.221227750860346,0.153846153846154,
-0.583326335743102));
#29582=CARTESIAN_POINT('Ctrl Pts',(-0.466969125257516,0.192307692307692,
-0.413698471057249));
#29583=CARTESIAN_POINT('Ctrl Pts',(-0.605737625154647,0.230769230769231,
-0.149301246402526));
#29584=CARTESIAN_POINT('Ctrl Pts',(-0.605736940333524,0.269230769230769,
0.14930101675222));
#29585=CARTESIAN_POINT('Ctrl Pts',(-0.466970187413293,0.307692307692308,
0.413699286558057));
#29586=CARTESIAN_POINT('Ctrl Pts',(-0.221225725123394,0.346153846153846,
0.583324484886018));
#29587=CARTESIAN_POINT('Ctrl Pts',(0.0751986583056162,0.384615384615385,
0.619316856641734));
#29588=CARTESIAN_POINT('Ctrl Pts',(0.354396045955746,0.423076923076923,
0.513431304005641));
#29589=CARTESIAN_POINT('Ctrl Pts',(0.55240551470084,0.461538461538462,0.289924779022985));
#29590=CARTESIAN_POINT('Ctrl Pts',(0.623865568763842,0.5,3.99584594159288E-16));
#29591=CARTESIAN_POINT('Ctrl Pts',(0.552405514700841,0.538461538461539,
-0.289924779022984));
#29592=CARTESIAN_POINT('Ctrl Pts',(0.354396045955747,0.576923076923077,
-0.513431304005641));
#29593=CARTESIAN_POINT('Ctrl Pts',(0.0751986583056171,0.615384615384616,
-0.619316856641735));
#29594=CARTESIAN_POINT('Ctrl Pts',(-0.221225725123393,0.653846153846154,
-0.583324484886017));
#29595=CARTESIAN_POINT('Ctrl Pts',(-0.466970187413293,0.692307692307693,
-0.413699286558058));
#29596=CARTESIAN_POINT('Ctrl Pts',(-0.605736940333523,0.730769230769231,
-0.149301016752221));
#29597=CARTESIAN_POINT('Ctrl Pts',(-0.605737625154647,0.769230769230769,
0.149301246402525));
#29598=CARTESIAN_POINT('Ctrl Pts',(-0.466969125257516,0.807692307692308,
0.41369847105725));
#29599=CARTESIAN_POINT('Ctrl Pts',(-0.221227750860347,0.846153846153846,
0.583326335743102));
#29600=CARTESIAN_POINT('Ctrl Pts',(0.0752027553952735,0.884615384615385,
0.619312950390957));
#29601=CARTESIAN_POINT('Ctrl Pts',(0.354387423761003,0.923076923076923,
0.513439446520879));
#29602=CARTESIAN_POINT('Ctrl Pts',(0.552422075024676,0.961538461538462,
0.289907779312462));
#29603=CARTESIAN_POINT('Ctrl Pts',(0.6,0.987179487179487,0.096664389341225));
#29604=CARTESIAN_POINT('Ctrl Pts',(0.6,1.,2.93915231795365E-16));
#29605=CARTESIAN_POINT('',(0.6,-1.22464679914735E-17,0.));
#29606=CARTESIAN_POINT('Origin',(0.5,0.,0.));
#29607=CARTESIAN_POINT('',(0.6,1.,2.93915231795365E-16));
#29608=CARTESIAN_POINT('Ctrl Pts',(0.6,1.22464679914735E-17,0.));
#29609=CARTESIAN_POINT('Ctrl Pts',(0.6,0.0128205128205128,-0.0966643893412244));
#29610=CARTESIAN_POINT('Ctrl Pts',(0.552422075024677,0.0384615384615385,
-0.289907779312461));
#29611=CARTESIAN_POINT('Ctrl Pts',(0.354387423761003,0.076923076923077,
-0.513439446520879));
#29612=CARTESIAN_POINT('Ctrl Pts',(0.0752027553952744,0.115384615384615,
-0.619312950390957));
#29613=CARTESIAN_POINT('Ctrl Pts',(-0.221227750860346,0.153846153846154,
-0.583326335743102));
#29614=CARTESIAN_POINT('Ctrl Pts',(-0.466969125257516,0.192307692307692,
-0.413698471057249));
#29615=CARTESIAN_POINT('Ctrl Pts',(-0.605737625154647,0.230769230769231,
-0.149301246402526));
#29616=CARTESIAN_POINT('Ctrl Pts',(-0.605736940333524,0.269230769230769,
0.14930101675222));
#29617=CARTESIAN_POINT('Ctrl Pts',(-0.466970187413293,0.307692307692308,
0.413699286558057));
#29618=CARTESIAN_POINT('Ctrl Pts',(-0.221225725123394,0.346153846153846,
0.583324484886018));
#29619=CARTESIAN_POINT('Ctrl Pts',(0.0751986583056162,0.384615384615385,
0.619316856641734));
#29620=CARTESIAN_POINT('Ctrl Pts',(0.354396045955746,0.423076923076923,
0.513431304005641));
#29621=CARTESIAN_POINT('Ctrl Pts',(0.55240551470084,0.461538461538462,0.289924779022985));
#29622=CARTESIAN_POINT('Ctrl Pts',(0.623865568763842,0.5,3.99584594159288E-16));
#29623=CARTESIAN_POINT('Ctrl Pts',(0.552405514700841,0.538461538461539,
-0.289924779022984));
#29624=CARTESIAN_POINT('Ctrl Pts',(0.354396045955747,0.576923076923077,
-0.513431304005641));
#29625=CARTESIAN_POINT('Ctrl Pts',(0.0751986583056171,0.615384615384616,
-0.619316856641735));
#29626=CARTESIAN_POINT('Ctrl Pts',(-0.221225725123393,0.653846153846154,
-0.583324484886017));
#29627=CARTESIAN_POINT('Ctrl Pts',(-0.466970187413293,0.692307692307693,
-0.413699286558058));
#29628=CARTESIAN_POINT('Ctrl Pts',(-0.605736940333523,0.730769230769231,
-0.149301016752221));
#29629=CARTESIAN_POINT('Ctrl Pts',(-0.605737625154647,0.769230769230769,
0.149301246402525));
#29630=CARTESIAN_POINT('Ctrl Pts',(-0.466969125257516,0.807692307692308,
0.41369847105725));
#29631=CARTESIAN_POINT('Ctrl Pts',(-0.221227750860347,0.846153846153846,
0.583326335743102));
#29632=CARTESIAN_POINT('Ctrl Pts',(0.0752027553952735,0.884615384615385,
0.619312950390957));
#29633=CARTESIAN_POINT('Ctrl Pts',(0.354387423761003,0.923076923076923,
0.513439446520879));
#29634=CARTESIAN_POINT('Ctrl Pts',(0.552422075024676,0.961538461538462,
0.289907779312462));
#29635=CARTESIAN_POINT('Ctrl Pts',(0.6,0.987179487179487,0.096664389341225));
#29636=CARTESIAN_POINT('Ctrl Pts',(0.6,1.,2.93915231795365E-16));
#29637=CARTESIAN_POINT('Origin',(0.5,1.,2.44929359829471E-16));
#29638=CARTESIAN_POINT('Origin',(0.5,1.,2.44929359829471E-16));
#29639=CARTESIAN_POINT('Origin',(0.5,1.44560289664734E-18,0.));
#36458=UNCERTAINTY_MEASURE_WITH_UNIT(LENGTH_MEASURE(0.001),#36483,
'DISTANCE_ACCURACY_VALUE',
'Maximum model space distance between geometric entities at asserted c
onnectivities');
#36463=UNCERTAINTY_MEASURE_WITH_UNIT(LENGTH_MEASURE(0.001),#36483,
'DISTANCE_ACCURACY_VALUE',
'Maximum model space distance between geometric entities at asserted c
onnectivities');
#36477=(
GEOMETRIC_REPRESENTATION_CONTEXT(3)
GLOBAL_UNCERTAINTY_ASSIGNED_CONTEXT((#36458))
GLOBAL_UNIT_ASSIGNED_CONTEXT((#36483,#36485,#36486))
REPRESENTATION_CONTEXT('','3D')
);
#36482=(
GEOMETRIC_REPRESENTATION_CONTEXT(3)
GLOBAL_UNCERTAINTY_ASSIGNED_CONTEXT((#36463))
GLOBAL_UNIT_ASSIGNED_CONTEXT((#36483,#36485,#36486))
REPRESENTATION_CONTEXT('','3D')
);
#36483=(
LENGTH_UNIT()
NAMED_UNIT(*)
SI_UNIT(.CENTI.,.METRE.)
);
#36485=(
NAMED_UNIT(*)
PLANE_ANGLE_UNIT()
SI_UNIT($,.RADIAN.)
);
#36486=(
NAMED_UNIT(*)
SI_UNIT($,.STERADIAN.)
SOLID_ANGLE_UNIT()
);
#36500=SHAPE_DEFINITION_REPRESENTATION(#36518,#36567);
#36518=PRODUCT_DEFINITION_SHAPE('',$,#36586);
#36567=SHAPE_REPRESENTATION('',(#10491),#36477);
#36572=PRODUCT_DEFINITION_CONTEXT('part definition',#36628,'design');
#36586=PRODUCT_DEFINITION('Compression spring','Compression spring',#36604,
#36572);
#36604=PRODUCT_DEFINITION_FORMATION('',$,#36643);
#36628=APPLICATION_CONTEXT(
'Core Data for Automotive Mechanical Design Process');
#36629=PRODUCT_CONTEXT('part definition',#36628,'mechanical');
#36643=PRODUCT('Compression spring','Compression spring',
'Reusable native Coil compression spring created and edited through Fu
sion UI. Mean diameter6mm, round wire1mm,2turns, overall free height5m
m; plain open ends. Axis+Y, initial wire centerY0, physical boundsY\X2\2212\X0\0.
5..4.5mm. Native parameters retain wire section when configuring worki
ng height4mm. No nonuniform body scaling or Boolean construction. Mate
rial temper, seats, stiffness, preload, buckling, fatigue and life not
 rated.',(#36629));
#36660=PRESENTATION_STYLE_ASSIGNMENT((#36674));
#36674=SURFACE_STYLE_USAGE(.BOTH.,#36688);
#36688=SURFACE_SIDE_STYLE('',(#36702));
#36702=SURFACE_STYLE_FILL_AREA(#36716);
#36716=FILL_AREA_STYLE('Spring gray',(#36730));
#36730=FILL_AREA_STYLE_COLOUR('Spring gray',#36744);
#36744=COLOUR_RGB('Spring gray',0.407843137254902,0.447058823529412,0.498039215686275);
ENDSEC;
END-ISO-10303-21;
